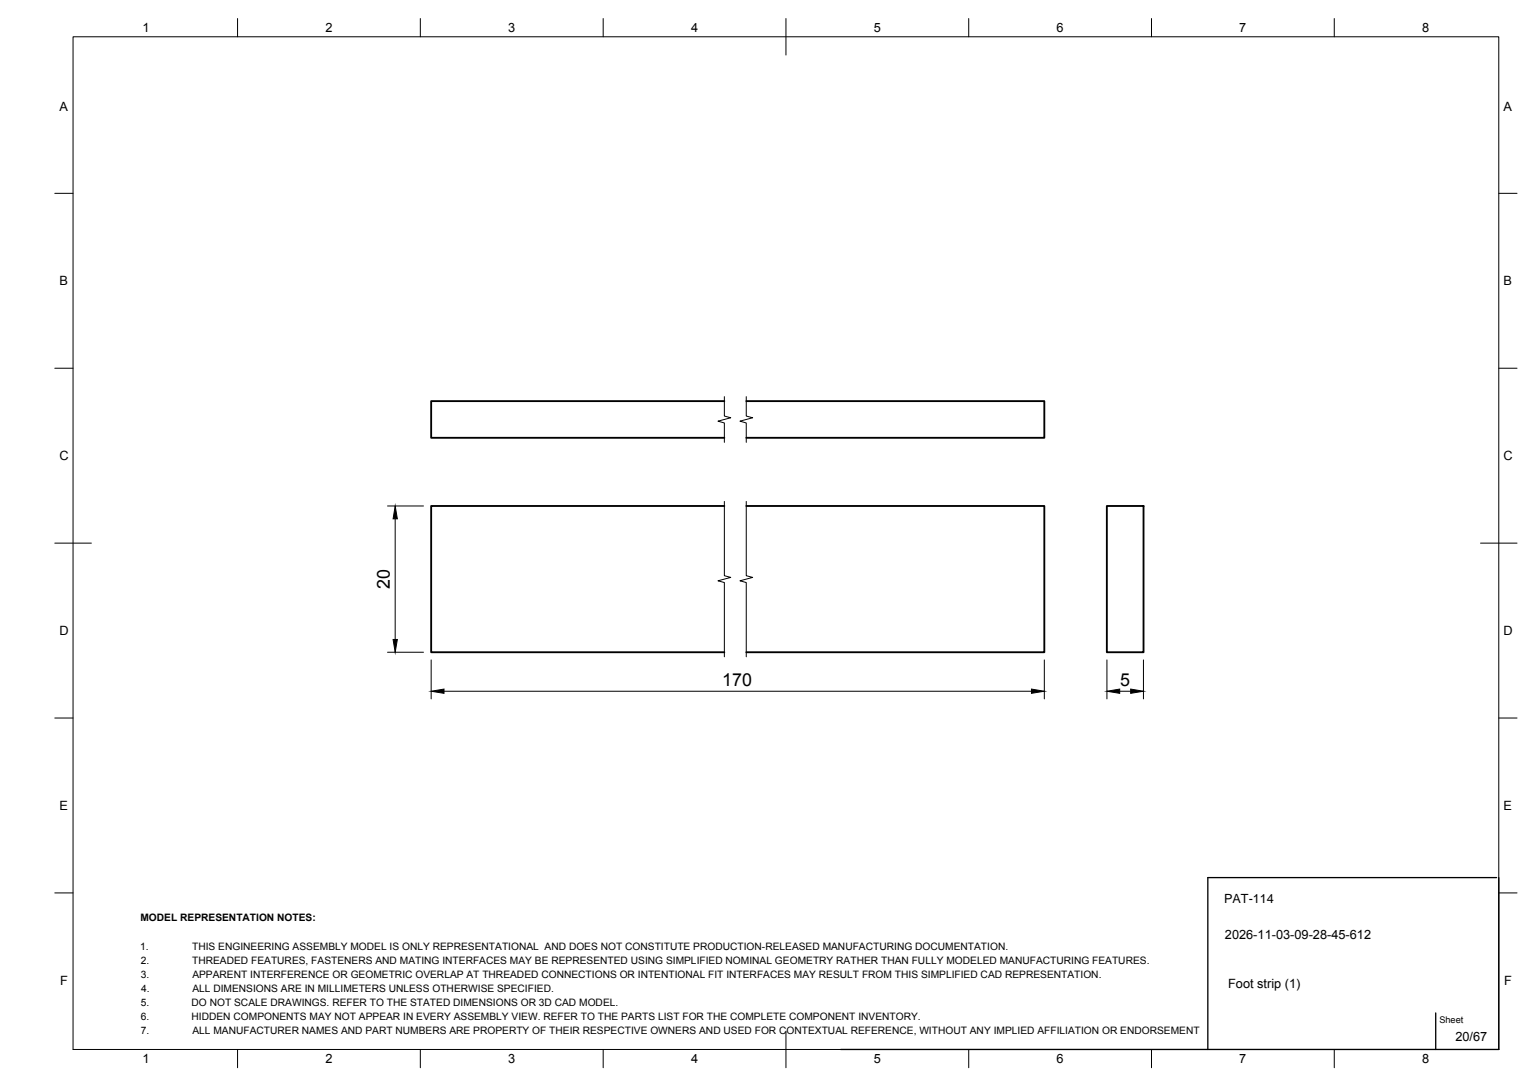
ISO-10303-21;
HEADER;
/* Generated by software containing ST-Developer
 * from STEP Tools, Inc. (www.steptools.com) 
 */

FILE_DESCRIPTION(
/* description */ ('Two-stage gear reducer in split housing'),
/* implementation_level */ '2;1');

FILE_NAME(
/* name */ 'Foot strip (1).step',
/* time_stamp */ '2026-10-28T03:22:31-07:00',
/* author */ (''),
/* organization */ (''),
/* preprocessor_version */ 'ST-DEVELOPER v20.2',
/* originating_system */ 'Autodesk Translation Framework v15.17.0.0',
/* authorisation */ '');

FILE_SCHEMA (('AUTOMOTIVE_DESIGN { 1 0 10303 214 3 1 1 }'));
ENDSEC;

DATA;
#10=MECHANICAL_DESIGN_GEOMETRIC_PRESENTATION_REPRESENTATION('',(#1249),#73366);
#1137=SHAPE_REPRESENTATION_RELATIONSHIP('SRR','None',#73624,#1193);
#1193=ADVANCED_BREP_SHAPE_REPRESENTATION('',(#1320),#73320);
#1249=STYLED_ITEM('',(#73974),#1320);
#1320=MANIFOLD_SOLID_BREP('Body1',#16137);
#1738=PLANE('',#17386);
#1739=PLANE('',#17387);
#1740=PLANE('',#17388);
#1741=PLANE('',#17389);
#1742=PLANE('',#17390);
#1743=PLANE('',#17391);
#2278=FACE_OUTER_BOUND('',#3335,.T.);
#2279=FACE_OUTER_BOUND('',#3336,.T.);
#2280=FACE_OUTER_BOUND('',#3337,.T.);
#2281=FACE_OUTER_BOUND('',#3338,.T.);
#2282=FACE_OUTER_BOUND('',#3339,.T.);
#2283=FACE_OUTER_BOUND('',#3340,.T.);
#3335=EDGE_LOOP('',(#11731,#11732,#11733,#11734));
#3336=EDGE_LOOP('',(#11735,#11736,#11737,#11738));
#3337=EDGE_LOOP('',(#11739,#11740,#11741,#11742));
#3338=EDGE_LOOP('',(#11743,#11744,#11745,#11746));
#3339=EDGE_LOOP('',(#11747,#11748,#11749,#11750));
#3340=EDGE_LOOP('',(#11751,#11752,#11753,#11754));
#4388=LINE('',#24091,#5412);
#4389=LINE('',#24093,#5413);
#4390=LINE('',#24095,#5414);
#4391=LINE('',#24096,#5415);
#4392=LINE('',#24099,#5416);
#4393=LINE('',#24101,#5417);
#4394=LINE('',#24102,#5418);
#4395=LINE('',#24105,#5419);
#4396=LINE('',#24107,#5420);
#4397=LINE('',#24108,#5421);
#4398=LINE('',#24110,#5422);
#4399=LINE('',#24111,#5423);
#5412=VECTOR('',#19940,1.);
#5413=VECTOR('',#19941,1.);
#5414=VECTOR('',#19942,1.);
#5415=VECTOR('',#19943,1.);
#5416=VECTOR('',#19946,1.);
#5417=VECTOR('',#19947,1.);
#5418=VECTOR('',#19948,1.);
#5419=VECTOR('',#19951,1.);
#5420=VECTOR('',#19952,1.);
#5421=VECTOR('',#19953,1.);
#5422=VECTOR('',#19956,1.);
#5423=VECTOR('',#19957,1.);
#7232=VERTEX_POINT('',#24089);
#7233=VERTEX_POINT('',#24090);
#7234=VERTEX_POINT('',#24092);
#7235=VERTEX_POINT('',#24094);
#7236=VERTEX_POINT('',#24098);
#7237=VERTEX_POINT('',#24100);
#7238=VERTEX_POINT('',#24104);
#7239=VERTEX_POINT('',#24106);
#8919=EDGE_CURVE('',#7232,#7233,#4388,.T.);
#8920=EDGE_CURVE('',#7233,#7234,#4389,.T.);
#8921=EDGE_CURVE('',#7235,#7234,#4390,.T.);
#8922=EDGE_CURVE('',#7232,#7235,#4391,.T.);
#8923=EDGE_CURVE('',#7236,#7232,#4392,.T.);
#8924=EDGE_CURVE('',#7237,#7235,#4393,.T.);
#8925=EDGE_CURVE('',#7236,#7237,#4394,.T.);
#8926=EDGE_CURVE('',#7238,#7236,#4395,.T.);
#8927=EDGE_CURVE('',#7239,#7237,#4396,.T.);
#8928=EDGE_CURVE('',#7238,#7239,#4397,.T.);
#8929=EDGE_CURVE('',#7233,#7238,#4398,.T.);
#8930=EDGE_CURVE('',#7234,#7239,#4399,.T.);
#11731=ORIENTED_EDGE('',*,*,#8919,.T.);
#11732=ORIENTED_EDGE('',*,*,#8920,.T.);
#11733=ORIENTED_EDGE('',*,*,#8921,.F.);
#11734=ORIENTED_EDGE('',*,*,#8922,.F.);
#11735=ORIENTED_EDGE('',*,*,#8923,.T.);
#11736=ORIENTED_EDGE('',*,*,#8922,.T.);
#11737=ORIENTED_EDGE('',*,*,#8924,.F.);
#11738=ORIENTED_EDGE('',*,*,#8925,.F.);
#11739=ORIENTED_EDGE('',*,*,#8926,.T.);
#11740=ORIENTED_EDGE('',*,*,#8925,.T.);
#11741=ORIENTED_EDGE('',*,*,#8927,.F.);
#11742=ORIENTED_EDGE('',*,*,#8928,.F.);
#11743=ORIENTED_EDGE('',*,*,#8929,.T.);
#11744=ORIENTED_EDGE('',*,*,#8928,.T.);
#11745=ORIENTED_EDGE('',*,*,#8930,.F.);
#11746=ORIENTED_EDGE('',*,*,#8920,.F.);
#11747=ORIENTED_EDGE('',*,*,#8930,.T.);
#11748=ORIENTED_EDGE('',*,*,#8927,.T.);
#11749=ORIENTED_EDGE('',*,*,#8924,.T.);
#11750=ORIENTED_EDGE('',*,*,#8921,.T.);
#11751=ORIENTED_EDGE('',*,*,#8929,.F.);
#11752=ORIENTED_EDGE('',*,*,#8919,.F.);
#11753=ORIENTED_EDGE('',*,*,#8923,.F.);
#11754=ORIENTED_EDGE('',*,*,#8926,.F.);
#15485=ADVANCED_FACE('',(#2278),#1738,.T.);
#15486=ADVANCED_FACE('',(#2279),#1739,.T.);
#15487=ADVANCED_FACE('',(#2280),#1740,.T.);
#15488=ADVANCED_FACE('',(#2281),#1741,.T.);
#15489=ADVANCED_FACE('',(#2282),#1742,.T.);
#15490=ADVANCED_FACE('',(#2283),#1743,.F.);
#16137=CLOSED_SHELL('',(#15485,#15486,#15487,#15488,#15489,#15490));
#17385=AXIS2_PLACEMENT_3D('',#24087,#19936,#19937);
#17386=AXIS2_PLACEMENT_3D('',#24088,#19938,#19939);
#17387=AXIS2_PLACEMENT_3D('',#24097,#19944,#19945);
#17388=AXIS2_PLACEMENT_3D('',#24103,#19949,#19950);
#17389=AXIS2_PLACEMENT_3D('',#24109,#19954,#19955);
#17390=AXIS2_PLACEMENT_3D('',#24112,#19958,#19959);
#17391=AXIS2_PLACEMENT_3D('',#24113,#19960,#19961);
#19936=DIRECTION('axis',(0.,0.,1.));
#19937=DIRECTION('refdir',(1.,0.,0.));
#19938=DIRECTION('center_axis',(0.,1.,0.));
#19939=DIRECTION('ref_axis',(-1.,0.,0.));
#19940=DIRECTION('',(-1.,0.,0.));
#19941=DIRECTION('',(0.,0.,1.));
#19942=DIRECTION('',(-1.,0.,0.));
#19943=DIRECTION('',(0.,0.,1.));
#19944=DIRECTION('center_axis',(1.,0.,0.));
#19945=DIRECTION('ref_axis',(0.,1.,0.));
#19946=DIRECTION('',(0.,1.,0.));
#19947=DIRECTION('',(0.,1.,0.));
#19948=DIRECTION('',(0.,0.,1.));
#19949=DIRECTION('center_axis',(0.,-1.,0.));
#19950=DIRECTION('ref_axis',(1.,0.,0.));
#19951=DIRECTION('',(1.,0.,0.));
#19952=DIRECTION('',(1.,0.,0.));
#19953=DIRECTION('',(0.,0.,1.));
#19954=DIRECTION('center_axis',(-1.,0.,0.));
#19955=DIRECTION('ref_axis',(0.,-1.,0.));
#19956=DIRECTION('',(0.,-1.,0.));
#19957=DIRECTION('',(0.,-1.,0.));
#19958=DIRECTION('center_axis',(0.,0.,1.));
#19959=DIRECTION('ref_axis',(1.,0.,0.));
#19960=DIRECTION('center_axis',(0.,0.,1.));
#19961=DIRECTION('ref_axis',(1.,0.,0.));
#24087=CARTESIAN_POINT('',(0.,0.,0.));
#24088=CARTESIAN_POINT('Origin',(18.5,8.5,-0.5));
#24089=CARTESIAN_POINT('',(18.5,8.5,-0.5));
#24090=CARTESIAN_POINT('',(16.5,8.5,-0.5));
#24091=CARTESIAN_POINT('',(18.5,8.5,-0.5));
#24092=CARTESIAN_POINT('',(16.5,8.5,0.));
#24093=CARTESIAN_POINT('',(16.5,8.5,-0.5));
#24094=CARTESIAN_POINT('',(18.5,8.5,0.));
#24095=CARTESIAN_POINT('',(18.5,8.5,0.));
#24096=CARTESIAN_POINT('',(18.5,8.5,-0.5));
#24097=CARTESIAN_POINT('Origin',(18.5,-8.5,-0.5));
#24098=CARTESIAN_POINT('',(18.5,-8.5,-0.5));
#24099=CARTESIAN_POINT('',(18.5,-8.5,-0.5));
#24100=CARTESIAN_POINT('',(18.5,-8.5,0.));
#24101=CARTESIAN_POINT('',(18.5,-8.5,0.));
#24102=CARTESIAN_POINT('',(18.5,-8.5,-0.5));
#24103=CARTESIAN_POINT('Origin',(16.5,-8.5,-0.5));
#24104=CARTESIAN_POINT('',(16.5,-8.5,-0.5));
#24105=CARTESIAN_POINT('',(16.5,-8.5,-0.5));
#24106=CARTESIAN_POINT('',(16.5,-8.5,0.));
#24107=CARTESIAN_POINT('',(16.5,-8.5,0.));
#24108=CARTESIAN_POINT('',(16.5,-8.5,-0.5));
#24109=CARTESIAN_POINT('Origin',(16.5,8.5,-0.5));
#24110=CARTESIAN_POINT('',(16.5,8.5,-0.5));
#24111=CARTESIAN_POINT('',(16.5,8.5,0.));
#24112=CARTESIAN_POINT('Origin',(17.5,0.,0.));
#24113=CARTESIAN_POINT('Origin',(17.5,0.,-0.5));
#73256=UNCERTAINTY_MEASURE_WITH_UNIT(LENGTH_MEASURE(0.001),#73367,
'DISTANCE_ACCURACY_VALUE',
'Maximum model space distance between geometric entities at asserted c
onnectivities');
#73302=UNCERTAINTY_MEASURE_WITH_UNIT(LENGTH_MEASURE(0.001),#73367,
'DISTANCE_ACCURACY_VALUE',
'Maximum model space distance between geometric entities at asserted c
onnectivities');
#73320=(
GEOMETRIC_REPRESENTATION_CONTEXT(3)
GLOBAL_UNCERTAINTY_ASSIGNED_CONTEXT((#73256))
GLOBAL_UNIT_ASSIGNED_CONTEXT((#73367,#73369,#73370))
REPRESENTATION_CONTEXT('','3D')
);
#73366=(
GEOMETRIC_REPRESENTATION_CONTEXT(3)
GLOBAL_UNCERTAINTY_ASSIGNED_CONTEXT((#73302))
GLOBAL_UNIT_ASSIGNED_CONTEXT((#73367,#73369,#73370))
REPRESENTATION_CONTEXT('','3D')
);
#73367=(
LENGTH_UNIT()
NAMED_UNIT(*)
SI_UNIT(.CENTI.,.METRE.)
);
#73369=(
NAMED_UNIT(*)
PLANE_ANGLE_UNIT()
SI_UNIT($,.RADIAN.)
);
#73370=(
NAMED_UNIT(*)
SI_UNIT($,.STERADIAN.)
SOLID_ANGLE_UNIT()
);
#73388=SHAPE_DEFINITION_REPRESENTATION(#73451,#73624);
#73451=PRODUCT_DEFINITION_SHAPE('',$,#73688);
#73624=SHAPE_REPRESENTATION('',(#17385),#73320);
#73670=PRODUCT_DEFINITION_CONTEXT('part definition',#73861,'design');
#73688=PRODUCT_DEFINITION('Foot strip (1)','Foot strip (1)',#73751,#73670);
#73751=PRODUCT_DEFINITION_FORMATION('',$,#73880);
#73861=APPLICATION_CONTEXT(
'Core Data for Automotive Mechanical Design Process');
#73862=PRODUCT_CONTEXT('part definition',#73861,'mechanical');
#73880=PRODUCT('Foot strip (1)','Foot strip (1)','Foot strip (1)',(#73862));
#73968=COLOUR_RGB('Light Blue',0.38,0.62,0.78);
#73969=FILL_AREA_STYLE_COLOUR('',#73968);
#73970=FILL_AREA_STYLE('',(#73969));
#73971=SURFACE_STYLE_FILL_AREA(#73970);
#73972=SURFACE_SIDE_STYLE('',(#73971));
#73973=SURFACE_STYLE_USAGE(.BOTH.,#73972);
#73974=PRESENTATION_STYLE_ASSIGNMENT((#73973));
ENDSEC;
END-ISO-10303-21;
